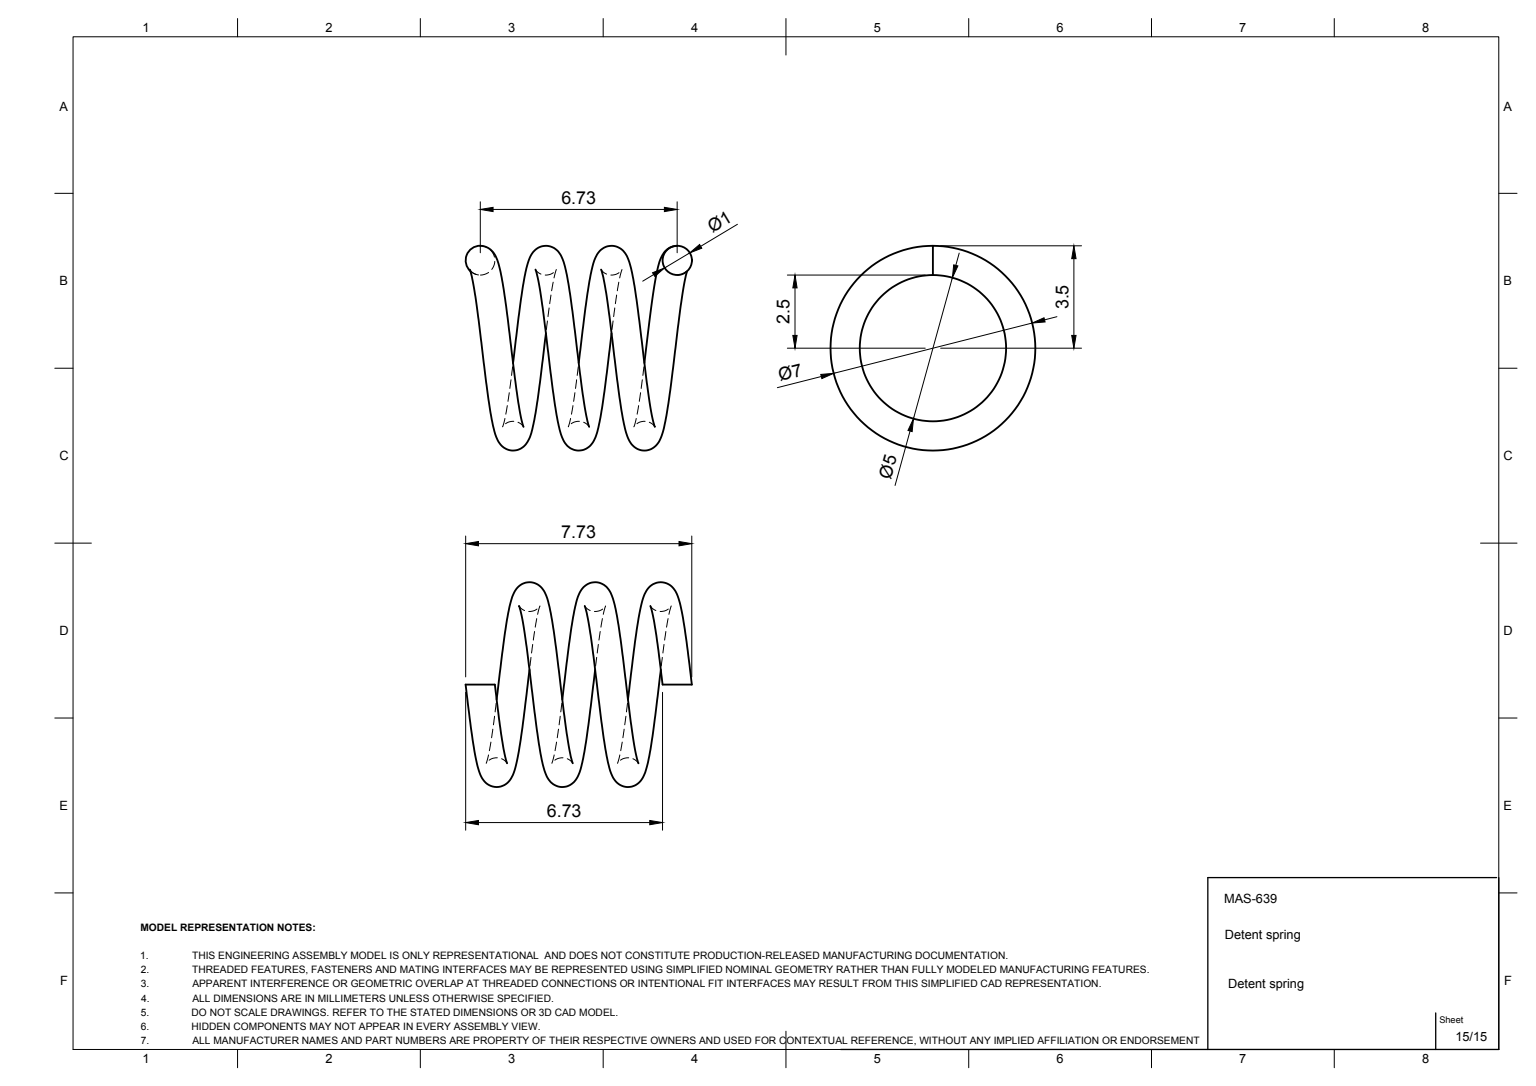
ISO-10303-21;
HEADER;
/* Generated by software containing ST-Developer
 * from STEP Tools, Inc. (www.steptools.com) 
 */

FILE_DESCRIPTION(
/* description */ ('Independent maintained push-to-latch/pull-to-reset mushroom-operator 
CAD. Two opposed spring-loaded ball detents in turned circular seats b
ias both travel stops; direct normally-closed bridge opens6mm when pre
ssed. Rounded palm/pull rim, captured head screw, removable detent clo
sures, native Coil spring families, insulated shared terminals and ord
inary machining features. Manual geometric states and ideal same-mater
ial spring-energy direction only; no electrical/safety certification, 
force/contact dynamics, wear, load or life rating. Requested blue/gray
 visual palette, not safety identification. External wiring/anchors an
d application engineering omitted.'),
/* implementation_level */ '2;1');

FILE_NAME(
/* name */ 'Detent spring.step',
/* time_stamp */ '2026-11-08T17:54:26-08:00',
/* author */ (''),
/* organization */ (''),
/* preprocessor_version */ 'ST-DEVELOPER v20.2',
/* originating_system */ 'Autodesk Translation Framework v15.17.0.0',
/* authorisation */ '');

FILE_SCHEMA (('AUTOMOTIVE_DESIGN { 1 0 10303 214 3 1 1 }'));
ENDSEC;

DATA;
#10=MECHANICAL_DESIGN_GEOMETRIC_PRESENTATION_REPRESENTATION('',(#202),#43980);
#168=SHAPE_REPRESENTATION_RELATIONSHIP('SRR','None',#44068,#185);
#185=ADVANCED_BREP_SHAPE_REPRESENTATION('',(#219),#43975);
#202=STYLED_ITEM('',(#44155),#219);
#219=MANIFOLD_SOLID_BREP('Body1',#11243);
#249=B_SPLINE_SURFACE_WITH_KNOTS('',3,3,((#35913,#35914,#35915,#35916,#35917,
#35918,#35919,#35920,#35921,#35922,#35923,#35924,#35925,#35926,#35927,#35928,
#35929,#35930,#35931,#35932,#35933,#35934,#35935,#35936,#35937,#35938,#35939,
#35940,#35941,#35942,#35943,#35944,#35945,#35946,#35947,#35948,#35949,#35950,
#35951,#35952,#35953),(#35954,#35955,#35956,#35957,#35958,#35959,#35960,
#35961,#35962,#35963,#35964,#35965,#35966,#35967,#35968,#35969,#35970,#35971,
#35972,#35973,#35974,#35975,#35976,#35977,#35978,#35979,#35980,#35981,#35982,
#35983,#35984,#35985,#35986,#35987,#35988,#35989,#35990,#35991,#35992,#35993,
#35994),(#35995,#35996,#35997,#35998,#35999,#36000,#36001,#36002,#36003,
#36004,#36005,#36006,#36007,#36008,#36009,#36010,#36011,#36012,#36013,#36014,
#36015,#36016,#36017,#36018,#36019,#36020,#36021,#36022,#36023,#36024,#36025,
#36026,#36027,#36028,#36029,#36030,#36031,#36032,#36033,#36034,#36035),
(#36036,#36037,#36038,#36039,#36040,#36041,#36042,#36043,#36044,#36045,
#36046,#36047,#36048,#36049,#36050,#36051,#36052,#36053,#36054,#36055,#36056,
#36057,#36058,#36059,#36060,#36061,#36062,#36063,#36064,#36065,#36066,#36067,
#36068,#36069,#36070,#36071,#36072,#36073,#36074,#36075,#36076),(#36077,
#36078,#36079,#36080,#36081,#36082,#36083,#36084,#36085,#36086,#36087,#36088,
#36089,#36090,#36091,#36092,#36093,#36094,#36095,#36096,#36097,#36098,#36099,
#36100,#36101,#36102,#36103,#36104,#36105,#36106,#36107,#36108,#36109,#36110,
#36111,#36112,#36113,#36114,#36115,#36116,#36117),(#36118,#36119,#36120,
#36121,#36122,#36123,#36124,#36125,#36126,#36127,#36128,#36129,#36130,#36131,
#36132,#36133,#36134,#36135,#36136,#36137,#36138,#36139,#36140,#36141,#36142,
#36143,#36144,#36145,#36146,#36147,#36148,#36149,#36150,#36151,#36152,#36153,
#36154,#36155,#36156,#36157,#36158),(#36159,#36160,#36161,#36162,#36163,
#36164,#36165,#36166,#36167,#36168,#36169,#36170,#36171,#36172,#36173,#36174,
#36175,#36176,#36177,#36178,#36179,#36180,#36181,#36182,#36183,#36184,#36185,
#36186,#36187,#36188,#36189,#36190,#36191,#36192,#36193,#36194,#36195,#36196,
#36197,#36198,#36199),(#36200,#36201,#36202,#36203,#36204,#36205,#36206,
#36207,#36208,#36209,#36210,#36211,#36212,#36213,#36214,#36215,#36216,#36217,
#36218,#36219,#36220,#36221,#36222,#36223,#36224,#36225,#36226,#36227,#36228,
#36229,#36230,#36231,#36232,#36233,#36234,#36235,#36236,#36237,#36238,#36239,
#36240),(#36241,#36242,#36243,#36244,#36245,#36246,#36247,#36248,#36249,
#36250,#36251,#36252,#36253,#36254,#36255,#36256,#36257,#36258,#36259,#36260,
#36261,#36262,#36263,#36264,#36265,#36266,#36267,#36268,#36269,#36270,#36271,
#36272,#36273,#36274,#36275,#36276,#36277,#36278,#36279,#36280,#36281),
(#36282,#36283,#36284,#36285,#36286,#36287,#36288,#36289,#36290,#36291,
#36292,#36293,#36294,#36295,#36296,#36297,#36298,#36299,#36300,#36301,#36302,
#36303,#36304,#36305,#36306,#36307,#36308,#36309,#36310,#36311,#36312,#36313,
#36314,#36315,#36316,#36317,#36318,#36319,#36320,#36321,#36322)),
 .UNSPECIFIED.,.T.,.F.,.F.,(4,1,1,1,1,1,1,4),(4,1,1,1,1,1,1,1,1,1,1,1,1,
1,1,1,1,1,1,1,1,1,1,1,1,1,1,1,1,1,1,1,1,1,1,1,1,1,4),(-3.14159265358979,
-2.24399475256414,-1.34639685153848,-0.448798950512828,0.448798950512828,
1.34639685153848,2.24399475256414,3.14159265358979),(0.,0.496040945303652,
0.992081890607303,1.48812283591095,1.98416378121461,2.48020472651826,2.97624567182191,
3.47228661712556,3.96832756242921,4.46436850773286,4.96040945303652,5.45645039834017,
5.95249134364382,6.44853228894747,6.94457323425112,7.44061417955477,7.93665512485842,
8.43269607016208,8.92873701546573,9.42477796076938,9.92081890607303,10.4168598513767,
10.9129007966803,11.408941741984,11.9049826872876,12.4010236325913,12.8970645778949,
13.3931055231986,13.8891464685022,14.3851874138059,14.8812283591095,15.3772693044132,
15.8733102497168,16.3693511950205,16.8653921403242,17.3614330856278,17.8574740309315,
18.3535149762351,18.8495559215388),.UNSPECIFIED.);
#442=PLANE('',#12051);
#443=PLANE('',#12052);
#947=FACE_OUTER_BOUND('',#1634,.T.);
#948=FACE_OUTER_BOUND('',#1635,.T.);
#949=FACE_OUTER_BOUND('',#1636,.T.);
#1634=EDGE_LOOP('',(#9337,#9338,#9339,#9340));
#1635=EDGE_LOOP('',(#9341));
#1636=EDGE_LOOP('',(#9342));
#1962=CIRCLE('',#12049,0.05);
#1963=CIRCLE('',#12050,0.05);
#2609=B_SPLINE_CURVE_WITH_KNOTS('',3,(#36326,#36327,#36328,#36329,#36330,
#36331,#36332,#36333,#36334,#36335,#36336,#36337,#36338,#36339,#36340,#36341,
#36342,#36343,#36344,#36345,#36346,#36347,#36348,#36349,#36350,#36351,#36352,
#36353,#36354,#36355,#36356,#36357,#36358,#36359,#36360,#36361,#36362,#36363,
#36364,#36365,#36366),.UNSPECIFIED.,.F.,.F.,(4,1,1,1,1,1,1,1,1,1,1,1,1,
1,1,1,1,1,1,1,1,1,1,1,1,1,1,1,1,1,1,1,1,1,1,1,1,1,4),(0.,0.496040945303652,
0.992081890607303,1.48812283591095,1.98416378121461,2.48020472651826,2.97624567182191,
3.47228661712556,3.96832756242921,4.46436850773286,4.96040945303652,5.45645039834017,
5.95249134364382,6.44853228894747,6.94457323425112,7.44061417955477,7.93665512485842,
8.43269607016208,8.92873701546573,9.42477796076938,9.92081890607303,10.4168598513767,
10.9129007966803,11.408941741984,11.9049826872876,12.4010236325913,12.8970645778949,
13.3931055231986,13.8891464685022,14.3851874138059,14.8812283591095,15.3772693044132,
15.8733102497168,16.3693511950205,16.8653921403242,17.3614330856278,17.8574740309315,
18.3535149762351,18.8495559215388),.UNSPECIFIED.);
#4918=VERTEX_POINT('',#36323);
#4919=VERTEX_POINT('',#36325);
#6438=EDGE_CURVE('',#4918,#4918,#1962,.T.);
#6439=EDGE_CURVE('',#4918,#4919,#2609,.T.);
#6440=EDGE_CURVE('',#4919,#4919,#1963,.T.);
#9337=ORIENTED_EDGE('',*,*,#6438,.T.);
#9338=ORIENTED_EDGE('',*,*,#6439,.T.);
#9339=ORIENTED_EDGE('',*,*,#6440,.F.);
#9340=ORIENTED_EDGE('',*,*,#6439,.F.);
#9341=ORIENTED_EDGE('',*,*,#6440,.T.);
#9342=ORIENTED_EDGE('',*,*,#6438,.F.);
#11072=ADVANCED_FACE('',(#947),#249,.T.);
#11073=ADVANCED_FACE('',(#948),#442,.F.);
#11074=ADVANCED_FACE('',(#949),#443,.T.);
#11243=CLOSED_SHELL('',(#11072,#11073,#11074));
#12048=AXIS2_PLACEMENT_3D('',#35912,#13951,#13952);
#12049=AXIS2_PLACEMENT_3D('',#36324,#13953,#13954);
#12050=AXIS2_PLACEMENT_3D('',#36367,#13955,#13956);
#12051=AXIS2_PLACEMENT_3D('',#36368,#13957,#13958);
#12052=AXIS2_PLACEMENT_3D('',#36369,#13959,#13960);
#13951=DIRECTION('axis',(0.,0.,1.));
#13952=DIRECTION('refdir',(1.,0.,0.));
#13953=DIRECTION('center_axis',(0.,0.,-1.));
#13954=DIRECTION('ref_axis',(-1.,0.,0.));
#13955=DIRECTION('center_axis',(7.34788079488412E-16,0.,-1.));
#13956=DIRECTION('ref_axis',(-1.,0.,-7.34788079488412E-16));
#13957=DIRECTION('center_axis',(-7.34788079488412E-16,0.,1.));
#13958=DIRECTION('ref_axis',(1.,0.,7.34788079488412E-16));
#13959=DIRECTION('center_axis',(0.,0.,1.));
#13960=DIRECTION('ref_axis',(1.,0.,0.));
#35912=CARTESIAN_POINT('',(0.,0.,0.));
#35913=CARTESIAN_POINT('Ctrl Pts',(0.35,-6.12323399573676E-18,0.));
#35914=CARTESIAN_POINT('Ctrl Pts',(0.35,0.00590530772593761,-0.0578714436187594));
#35915=CARTESIAN_POINT('Ctrl Pts',(0.320737036978914,0.0177159231778128,
-0.173548309605457));
#35916=CARTESIAN_POINT('Ctrl Pts',(0.199460245847326,0.0354318463556257,
-0.305323295892745));
#35917=CARTESIAN_POINT('Ctrl Pts',(0.0301195604177668,0.0531477695334385,
-0.363416175774699));
#35918=CARTESIAN_POINT('Ctrl Pts',(-0.146502340124411,0.0708636927112515,
-0.333985996548453));
#35919=CARTESIAN_POINT('Ctrl Pts',(-0.287770405730312,0.088579615889064,
-0.223981002451209));
#35920=CARTESIAN_POINT('Ctrl Pts',(-0.359728502950795,0.106295539066877,
-0.0600284421673934));
#35921=CARTESIAN_POINT('Ctrl Pts',(-0.344906058802126,0.12401146224469,
0.118406781736645));
#35922=CARTESIAN_POINT('Ctrl Pts',(-0.247005954023888,0.141727385422503,
0.268319590417229));
#35923=CARTESIAN_POINT('Ctrl Pts',(-0.0895198614025972,0.159443308600316,
0.353506441262074));
#35924=CARTESIAN_POINT('Ctrl Pts',(0.0895288995299922,0.177159231778128,
0.353541847300449));
#35925=CARTESIAN_POINT('Ctrl Pts',(0.246980934267327,0.194875154955941,
0.268292799062886));
#35926=CARTESIAN_POINT('Ctrl Pts',(0.344941099461226,0.212591078133754,
0.118418424896554));
#35927=CARTESIAN_POINT('Ctrl Pts',(0.359691482037638,0.230307001311567,
-0.0600218865157286));
#35928=CARTESIAN_POINT('Ctrl Pts',(0.287800848035351,0.248022924489379,
-0.22400439780941));
#35929=CARTESIAN_POINT('Ctrl Pts',(0.146484276133641,0.265738847667193,
-0.33395050615258));
#35930=CARTESIAN_POINT('Ctrl Pts',(-0.0301168255445678,0.283454770845005,
-0.363456018331913));
#35931=CARTESIAN_POINT('Ctrl Pts',(-0.199452865725669,0.301170694022818,
-0.305285338376046));
#35932=CARTESIAN_POINT('Ctrl Pts',(-0.320745536260988,0.318886617200631,
-0.173578803829894));
#35933=CARTESIAN_POINT('Ctrl Pts',(-0.364665029422868,0.336602540378444,
-2.32705416708787E-16));
#35934=CARTESIAN_POINT('Ctrl Pts',(-0.320745536260988,0.354318463556256,
0.173578803829895));
#35935=CARTESIAN_POINT('Ctrl Pts',(-0.199452865725669,0.37203438673407,
0.305285338376046));
#35936=CARTESIAN_POINT('Ctrl Pts',(-0.0301168255445679,0.389750309911882,
0.363456018331913));
#35937=CARTESIAN_POINT('Ctrl Pts',(0.146484276133641,0.407466233089696,
0.33395050615258));
#35938=CARTESIAN_POINT('Ctrl Pts',(0.287800848035351,0.425182156267507,
0.224004397809409));
#35939=CARTESIAN_POINT('Ctrl Pts',(0.359691482037638,0.442898079445321,
0.0600218865157286));
#35940=CARTESIAN_POINT('Ctrl Pts',(0.344941099461226,0.460614002623134,
-0.118418424896554));
#35941=CARTESIAN_POINT('Ctrl Pts',(0.246980934267327,0.478329925800947,
-0.268292799062886));
#35942=CARTESIAN_POINT('Ctrl Pts',(0.0895288995299929,0.49604584897876,
-0.353541847300449));
#35943=CARTESIAN_POINT('Ctrl Pts',(-0.0895198614025975,0.513761772156572,
-0.353506441262075));
#35944=CARTESIAN_POINT('Ctrl Pts',(-0.247005954023888,0.531477695334385,
-0.268319590417228));
#35945=CARTESIAN_POINT('Ctrl Pts',(-0.344906058802126,0.549193618512198,
-0.118406781736645));
#35946=CARTESIAN_POINT('Ctrl Pts',(-0.359728502950795,0.56690954169001,
0.0600284421673935));
#35947=CARTESIAN_POINT('Ctrl Pts',(-0.287770405730312,0.584625464867824,
0.223981002451209));
#35948=CARTESIAN_POINT('Ctrl Pts',(-0.146502340124411,0.602341388045636,
0.333985996548453));
#35949=CARTESIAN_POINT('Ctrl Pts',(0.0301195604177669,0.62005731122345,
0.3634161757747));
#35950=CARTESIAN_POINT('Ctrl Pts',(0.199460245847326,0.637773234401262,
0.305323295892745));
#35951=CARTESIAN_POINT('Ctrl Pts',(0.320737036978914,0.655489157579075,
0.173548309605457));
#35952=CARTESIAN_POINT('Ctrl Pts',(0.35,0.66729977303095,0.0578714436187596));
#35953=CARTESIAN_POINT('Ctrl Pts',(0.35,0.673205080756888,2.57175827820944E-16));
#35954=CARTESIAN_POINT('Ctrl Pts',(0.35,-0.0149599650170943,0.));
#35955=CARTESIAN_POINT('Ctrl Pts',(0.35,-0.00905465729115664,-0.0578939412128541));
#35956=CARTESIAN_POINT('Ctrl Pts',(0.320737127540777,0.00275595816071859,
-0.17353420038403));
#35957=CARTESIAN_POINT('Ctrl Pts',(0.199462254474698,0.0204718813385314,
-0.305334734920036));
#35958=CARTESIAN_POINT('Ctrl Pts',(0.0301198482341514,0.0381878045163443,
-0.363411053172193));
#35959=CARTESIAN_POINT('Ctrl Pts',(-0.146504814797102,0.0559037276941571,
-0.33399283744356));
#35960=CARTESIAN_POINT('Ctrl Pts',(-0.287768683388874,0.0736196508719699,
-0.223978927605389));
#35961=CARTESIAN_POINT('Ctrl Pts',(-0.359733999999531,0.0913355740497829,
-0.060029831390249));
#35962=CARTESIAN_POINT('Ctrl Pts',(-0.344904107829491,0.109051497227595,
0.118406345723654));
#35963=CARTESIAN_POINT('Ctrl Pts',(-0.247009698820708,0.126767420405409,
0.268323507761981));
#35964=CARTESIAN_POINT('Ctrl Pts',(-0.0895193547402367,0.144483343583221,
0.353504534892372));
#35965=CARTESIAN_POINT('Ctrl Pts',(0.0895302448190081,0.162199266761034,
0.353547145096981));
#35966=CARTESIAN_POINT('Ctrl Pts',(0.246979562985841,0.179915189938847,
0.268291322927849));
#35967=CARTESIAN_POINT('Ctrl Pts',(0.344946301010151,0.19763111311666,0.118420201706933));
#35968=CARTESIAN_POINT('Ctrl Pts',(0.35968948216843,0.215347036294473,-0.0600215483887705));
#35969=CARTESIAN_POINT('Ctrl Pts',(0.287805188713831,0.233062959472285,
-0.224007779090794));
#35970=CARTESIAN_POINT('Ctrl Pts',(0.14648346160033,0.250778882650098,-0.333948647665377));
#35971=CARTESIAN_POINT('Ctrl Pts',(-0.0301172799130791,0.268494805827911,
-0.363461501186809));
#35972=CARTESIAN_POINT('Ctrl Pts',(-0.199451756376582,0.286210729005724,
-0.305283640177881));
#35973=CARTESIAN_POINT('Ctrl Pts',(-0.320750374264358,0.303926652183536,
-0.173581422140521));
#35974=CARTESIAN_POINT('Ctrl Pts',(-0.364663001235008,0.32164257536135,
-2.44953070219776E-16));
#35975=CARTESIAN_POINT('Ctrl Pts',(-0.320750374264359,0.339358498539162,
0.173581422140521));
#35976=CARTESIAN_POINT('Ctrl Pts',(-0.199451756376583,0.357074421716976,
0.305283640177881));
#35977=CARTESIAN_POINT('Ctrl Pts',(-0.0301172799130792,0.374790344894787,
0.363461501186809));
#35978=CARTESIAN_POINT('Ctrl Pts',(0.14648346160033,0.392506268072602,0.333948647665377));
#35979=CARTESIAN_POINT('Ctrl Pts',(0.287805188713831,0.410222191250413,
0.224007779090794));
#35980=CARTESIAN_POINT('Ctrl Pts',(0.35968948216843,0.427938114428227,0.0600215483887707));
#35981=CARTESIAN_POINT('Ctrl Pts',(0.344946301010151,0.445654037606039,
-0.118420201706934));
#35982=CARTESIAN_POINT('Ctrl Pts',(0.246979562985841,0.463369960783852,
-0.268291322927849));
#35983=CARTESIAN_POINT('Ctrl Pts',(0.0895302448190086,0.481085883961665,
-0.353547145096981));
#35984=CARTESIAN_POINT('Ctrl Pts',(-0.0895193547402369,0.498801807139478,
-0.353504534892371));
#35985=CARTESIAN_POINT('Ctrl Pts',(-0.247009698820707,0.516517730317291,
-0.268323507761982));
#35986=CARTESIAN_POINT('Ctrl Pts',(-0.344904107829491,0.534233653495103,
-0.118406345723654));
#35987=CARTESIAN_POINT('Ctrl Pts',(-0.359733999999531,0.551949576672917,
0.0600298313902493));
#35988=CARTESIAN_POINT('Ctrl Pts',(-0.287768683388874,0.569665499850729,
0.223978927605389));
#35989=CARTESIAN_POINT('Ctrl Pts',(-0.146504814797102,0.587381423028543,
0.333992837443561));
#35990=CARTESIAN_POINT('Ctrl Pts',(0.0301198482341516,0.605097346206355,
0.363411053172192));
#35991=CARTESIAN_POINT('Ctrl Pts',(0.199462254474698,0.622813269384167,
0.305334734920036));
#35992=CARTESIAN_POINT('Ctrl Pts',(0.320737127540777,0.640529192561981,
0.17353420038403));
#35993=CARTESIAN_POINT('Ctrl Pts',(0.35,0.652339808013856,0.0578939412128544));
#35994=CARTESIAN_POINT('Ctrl Pts',(0.35,0.658245115739793,2.57175827820944E-16));
#35995=CARTESIAN_POINT('Ctrl Pts',(0.335708111401436,-0.0447458605757917,
0.));
#35996=CARTESIAN_POINT('Ctrl Pts',(0.335708111401436,-0.0388405528498541,
-0.0554977928230549));
#35997=CARTESIAN_POINT('Ctrl Pts',(0.307640028870999,-0.0270299373979789,
-0.166468247501657));
#35998=CARTESIAN_POINT('Ctrl Pts',(0.191314552514196,-0.00931401422016608,
-0.292850380259684));
#35999=CARTESIAN_POINT('Ctrl Pts',(0.0288895245544089,0.00840190895764677,
-0.348578849160588));
#36000=CARTESIAN_POINT('Ctrl Pts',(-0.140518910052752,0.0261178321354596,
-0.32034482131761));
#36001=CARTESIAN_POINT('Ctrl Pts',(-0.276020404510637,0.0438337553132723,
-0.214835940639136));
#36002=CARTESIAN_POINT('Ctrl Pts',(-0.345036788048542,0.0615496784910853,
-0.0575765924801678));
#36003=CARTESIAN_POINT('Ctrl Pts',(-0.330823089198529,0.0792656016688981,
0.113571967147225));
#36004=CARTESIAN_POINT('Ctrl Pts',(-0.236917968165966,0.0969815248467109,
0.257361203462888));
#36005=CARTESIAN_POINT('Ctrl Pts',(-0.0858646474450097,0.114697448024524,
0.339072263044565));
#36006=CARTESIAN_POINT('Ctrl Pts',(0.0858724496913478,0.132413371202337,
0.33910285135484));
#36007=CARTESIAN_POINT('Ctrl Pts',(0.236896364680631,0.150129294380149,
0.257338030560792));
#36008=CARTESIAN_POINT('Ctrl Pts',(0.330853351222059,0.167845217557962,
0.113582099143669));
#36009=CARTESIAN_POINT('Ctrl Pts',(0.34500478782966,0.185561140735775,-0.0575711130196162));
#36010=CARTESIAN_POINT('Ctrl Pts',(0.276046765897809,0.203277063913588,
-0.214855826894537));
#36011=CARTESIAN_POINT('Ctrl Pts',(0.140503123221668,0.220992987091401,
-0.320314851940556));
#36012=CARTESIAN_POINT('Ctrl Pts',(-0.0288868234010755,0.238708910269214,
-0.348612100831537));
#36013=CARTESIAN_POINT('Ctrl Pts',(-0.191308933142308,0.256424833447026,
-0.292820121666851));
#36014=CARTESIAN_POINT('Ctrl Pts',(-0.307645959021329,0.274140756624839,
-0.166489667090601));
#36015=CARTESIAN_POINT('Ctrl Pts',(-0.349775258797716,0.291856679802652,
-1.83714802664832E-16));
#36016=CARTESIAN_POINT('Ctrl Pts',(-0.307645959021329,0.309572602980465,
0.166489667090601));
#36017=CARTESIAN_POINT('Ctrl Pts',(-0.191308933142307,0.327288526158277,
0.292820121666851));
#36018=CARTESIAN_POINT('Ctrl Pts',(-0.0288868234010758,0.345004449336091,
0.348612100831537));
#36019=CARTESIAN_POINT('Ctrl Pts',(0.140503123221668,0.362720372513903,
0.320314851940556));
#36020=CARTESIAN_POINT('Ctrl Pts',(0.27604676589781,0.380436295691716,0.214855826894537));
#36021=CARTESIAN_POINT('Ctrl Pts',(0.34500478782966,0.398152218869529,0.0575711130196162));
#36022=CARTESIAN_POINT('Ctrl Pts',(0.330853351222058,0.415868142047341,
-0.113582099143669));
#36023=CARTESIAN_POINT('Ctrl Pts',(0.236896364680631,0.433584065225155,
-0.257338030560792));
#36024=CARTESIAN_POINT('Ctrl Pts',(0.0858724496913482,0.451299988402968,
-0.33910285135484));
#36025=CARTESIAN_POINT('Ctrl Pts',(-0.0858646474450095,0.46901591158078,
-0.339072263044565));
#36026=CARTESIAN_POINT('Ctrl Pts',(-0.236917968165967,0.486731834758593,
-0.257361203462888));
#36027=CARTESIAN_POINT('Ctrl Pts',(-0.330823089198529,0.504447757936406,
-0.113571967147225));
#36028=CARTESIAN_POINT('Ctrl Pts',(-0.345036788048542,0.522163681114218,
0.0575765924801677));
#36029=CARTESIAN_POINT('Ctrl Pts',(-0.276020404510636,0.539879604292032,
0.214835940639137));
#36030=CARTESIAN_POINT('Ctrl Pts',(-0.140518910052752,0.557595527469844,
0.320344821317609));
#36031=CARTESIAN_POINT('Ctrl Pts',(0.0288895245544092,0.575311450647657,
0.348578849160589));
#36032=CARTESIAN_POINT('Ctrl Pts',(0.191314552514196,0.59302737382547,0.292850380259683));
#36033=CARTESIAN_POINT('Ctrl Pts',(0.307640028870999,0.610743297003283,
0.166468247501657));
#36034=CARTESIAN_POINT('Ctrl Pts',(0.335708111401436,0.622553912455158,
0.0554977928230551));
#36035=CARTESIAN_POINT('Ctrl Pts',(0.335708111401436,0.628459220181096,
2.46674318445343E-16));
#36036=CARTESIAN_POINT('Ctrl Pts',(0.287271575555009,-0.0557889266101467,
0.));
#36037=CARTESIAN_POINT('Ctrl Pts',(0.287271575555009,-0.0498836188842091,
-0.0475015952121335));
#36038=CARTESIAN_POINT('Ctrl Pts',(0.263253248344736,-0.0380730034323339,
-0.142442953697593));
#36039=CARTESIAN_POINT('Ctrl Pts',(0.163712356953626,-0.020357080254521,
-0.250603083626219));
#36040=CARTESIAN_POINT('Ctrl Pts',(0.0247214371762577,-0.00264115707670821,
-0.298282769894969));
#36041=CARTESIAN_POINT('Ctrl Pts',(-0.120245826277052,0.0150747661011046,
-0.27412830773178));
#36042=CARTESIAN_POINT('Ctrl Pts',(-0.236194861111183,0.0327906892789176,
-0.183838021283139));
#36043=CARTESIAN_POINT('Ctrl Pts',(-0.295257011496817,0.0505066124567302,
-0.0492700305779588));
#36044=CARTESIAN_POINT('Ctrl Pts',(-0.283090408491503,0.0682225356345432,
0.0971853955774754));
#36045=CARTESIAN_POINT('Ctrl Pts',(-0.202736892426251,0.0859384588123559,
0.220230628323799));
#36046=CARTESIAN_POINT('Ctrl Pts',(-0.0734757000535192,0.103654381990169,
0.290149399582528));
#36047=CARTESIAN_POINT('Ctrl Pts',(0.0734832917947263,0.121370305167982,
0.290179134787802));
#36048=CARTESIAN_POINT('Ctrl Pts',(0.202715877612707,0.139086228345794,
0.220208133442515));
#36049=CARTESIAN_POINT('Ctrl Pts',(0.283119838964945,0.156802151523607,
0.0971951592678911));
#36050=CARTESIAN_POINT('Ctrl Pts',(0.295225923420481,0.17451807470142,-0.0492644880639345));
#36051=CARTESIAN_POINT('Ctrl Pts',(0.236220415317673,0.192233997879233,
-0.183857734680427));
#36052=CARTESIAN_POINT('Ctrl Pts',(0.120230691703391,0.209949921057046,
-0.274098363237872));
#36053=CARTESIAN_POINT('Ctrl Pts',(-0.0247192080583375,0.227665844234859,
-0.298316465071458));
#36054=CARTESIAN_POINT('Ctrl Pts',(-0.16370600748086,0.245381767412672,
-0.250570698506515));
#36055=CARTESIAN_POINT('Ctrl Pts',(-0.263260669021949,0.263097690590484,
-0.142469549414193));
#36056=CARTESIAN_POINT('Ctrl Pts',(-0.299308088749296,0.280813613768297,
4.89906140439551E-17));
#36057=CARTESIAN_POINT('Ctrl Pts',(-0.263260669021949,0.29852953694611,
0.142469549414192));
#36058=CARTESIAN_POINT('Ctrl Pts',(-0.163706007480861,0.316245460123924,
0.250570698506515));
#36059=CARTESIAN_POINT('Ctrl Pts',(-0.0247192080583377,0.333961383301735,
0.298316465071458));
#36060=CARTESIAN_POINT('Ctrl Pts',(0.120230691703391,0.351677306479549,
0.274098363237873));
#36061=CARTESIAN_POINT('Ctrl Pts',(0.236220415317673,0.369393229657361,
0.183857734680427));
#36062=CARTESIAN_POINT('Ctrl Pts',(0.295225923420481,0.387109152835174,
0.0492644880639345));
#36063=CARTESIAN_POINT('Ctrl Pts',(0.283119838964945,0.404825076012987,
-0.0971951592678911));
#36064=CARTESIAN_POINT('Ctrl Pts',(0.202715877612707,0.4225409991908,-0.220208133442515));
#36065=CARTESIAN_POINT('Ctrl Pts',(0.0734832917947267,0.440256922368613,
-0.290179134787802));
#36066=CARTESIAN_POINT('Ctrl Pts',(-0.0734757000535193,0.457972845546425,
-0.290149399582527));
#36067=CARTESIAN_POINT('Ctrl Pts',(-0.202736892426251,0.47568876872424,
-0.220230628323799));
#36068=CARTESIAN_POINT('Ctrl Pts',(-0.283090408491504,0.493404691902051,
-0.0971853955774754));
#36069=CARTESIAN_POINT('Ctrl Pts',(-0.295257011496816,0.511120615079865,
0.0492700305779587));
#36070=CARTESIAN_POINT('Ctrl Pts',(-0.236194861111183,0.528836538257677,
0.183838021283139));
#36071=CARTESIAN_POINT('Ctrl Pts',(-0.120245826277051,0.54655246143549,
0.27412830773178));
#36072=CARTESIAN_POINT('Ctrl Pts',(0.0247214371762577,0.564268384613303,
0.298282769894969));
#36073=CARTESIAN_POINT('Ctrl Pts',(0.163712356953627,0.581984307791115,
0.250603083626218));
#36074=CARTESIAN_POINT('Ctrl Pts',(0.263253248344736,0.599700230968929,
0.142442953697593));
#36075=CARTESIAN_POINT('Ctrl Pts',(0.287271575555009,0.611510846420803,
0.0475015952121336));
#36076=CARTESIAN_POINT('Ctrl Pts',(0.287271575555009,0.617416154146741,
2.11083729293675E-16));
#36077=CARTESIAN_POINT('Ctrl Pts',(0.2483964525207,-0.0248377821418625,
0.));
#36078=CARTESIAN_POINT('Ctrl Pts',(0.2483964525207,-0.0189324744159249,
-0.0410748300994032));
#36079=CARTESIAN_POINT('Ctrl Pts',(0.227628419209138,-0.00712185896404963,
-0.123165932150964));
#36080=CARTESIAN_POINT('Ctrl Pts',(0.141558052308102,0.0105940642137631,
-0.216690850682477));
#36081=CARTESIAN_POINT('Ctrl Pts',(0.0213760183023638,0.0283099873915761,
-0.257917233510476));
#36082=CARTESIAN_POINT('Ctrl Pts',(-0.103973673673943,0.0460259105693889,
-0.237032228868884));
#36083=CARTESIAN_POINT('Ctrl Pts',(-0.204231604209003,0.0637418337472016,
-0.158959949419166));
#36084=CARTESIAN_POINT('Ctrl Pts',(-0.255301599773748,0.0814577569250147,
-0.0426026337570547));
#36085=CARTESIAN_POINT('Ctrl Pts',(-0.244780981522273,0.0991736801028273,
0.0840337218647635));
#36086=CARTESIAN_POINT('Ctrl Pts',(-0.175301687703595,0.11688960328064,
0.190428088650001));
#36087=CARTESIAN_POINT('Ctrl Pts',(-0.063532544489394,0.134605526458453,
0.250884715042728));
#36088=CARTESIAN_POINT('Ctrl Pts',(0.0635392244753556,0.152321449636266,
0.250910876008833));
#36089=CARTESIAN_POINT('Ctrl Pts',(0.175283197378719,0.170037372814079,
0.190408301232517));
#36090=CARTESIAN_POINT('Ctrl Pts',(0.244806875770799,0.187753295991892,
0.0840423024059766));
#36091=CARTESIAN_POINT('Ctrl Pts',(0.255274250740611,0.205469219169704,
-0.0425977334636045));
#36092=CARTESIAN_POINT('Ctrl Pts',(0.204254078740494,0.223185142347517,
-0.158977335668398));
#36093=CARTESIAN_POINT('Ctrl Pts',(0.103960381877751,0.24090106552533,-0.23700579360409));
#36094=CARTESIAN_POINT('Ctrl Pts',(-0.0213741012368434,0.258616988703143,
-0.25794703087359));
#36095=CARTESIAN_POINT('Ctrl Pts',(-0.141552367454289,0.276332911880956,
-0.216662028058088));
#36096=CARTESIAN_POINT('Ctrl Pts',(-0.227635132018289,0.294048835058769,
-0.123189972933852));
#36097=CARTESIAN_POINT('Ctrl Pts',(-0.25880399389923,0.311764758236581,
-1.22476535109888E-17));
#36098=CARTESIAN_POINT('Ctrl Pts',(-0.227635132018289,0.329480681414395,
0.123189972933851));
#36099=CARTESIAN_POINT('Ctrl Pts',(-0.141552367454289,0.347196604592207,
0.216662028058088));
#36100=CARTESIAN_POINT('Ctrl Pts',(-0.0213741012368437,0.364912527770019,
0.257947030873589));
#36101=CARTESIAN_POINT('Ctrl Pts',(0.103960381877751,0.382628450947834,
0.23700579360409));
#36102=CARTESIAN_POINT('Ctrl Pts',(0.204254078740494,0.400344374125644,
0.158977335668397));
#36103=CARTESIAN_POINT('Ctrl Pts',(0.255274250740611,0.418060297303459,
0.0425977334636048));
#36104=CARTESIAN_POINT('Ctrl Pts',(0.244806875770799,0.435776220481271,
-0.0840423024059769));
#36105=CARTESIAN_POINT('Ctrl Pts',(0.175283197378719,0.453492143659084,
-0.190408301232516));
#36106=CARTESIAN_POINT('Ctrl Pts',(0.0635392244753558,0.471208066836898,
-0.250910876008834));
#36107=CARTESIAN_POINT('Ctrl Pts',(-0.063532544489394,0.488923990014709,
-0.250884715042728));
#36108=CARTESIAN_POINT('Ctrl Pts',(-0.175301687703595,0.506639913192522,
-0.190428088650001));
#36109=CARTESIAN_POINT('Ctrl Pts',(-0.244780981522273,0.524355836370335,
-0.0840337218647634));
#36110=CARTESIAN_POINT('Ctrl Pts',(-0.255301599773748,0.542071759548147,
0.0426026337570547));
#36111=CARTESIAN_POINT('Ctrl Pts',(-0.204231604209003,0.559787682725961,
0.158959949419166));
#36112=CARTESIAN_POINT('Ctrl Pts',(-0.103973673673943,0.577503605903774,
0.237032228868883));
#36113=CARTESIAN_POINT('Ctrl Pts',(0.0213760183023641,0.595219529081586,
0.257917233510476));
#36114=CARTESIAN_POINT('Ctrl Pts',(0.141558052308102,0.6129354522594,0.216690850682477));
#36115=CARTESIAN_POINT('Ctrl Pts',(0.227628419209138,0.630651375437212,
0.123165932150964));
#36116=CARTESIAN_POINT('Ctrl Pts',(0.2483964525207,0.642461990889088,0.0410748300994034));
#36117=CARTESIAN_POINT('Ctrl Pts',(0.2483964525207,0.648367298615025,1.8251875229942E-16));
#36118=CARTESIAN_POINT('Ctrl Pts',(0.248462856117505,0.024811377463635,
0.));
#36119=CARTESIAN_POINT('Ctrl Pts',(0.248462856117505,0.0307166851895726,
-0.0410773426135567));
#36120=CARTESIAN_POINT('Ctrl Pts',(0.227689236819528,0.0425273006414479,
-0.123204168627986));
#36121=CARTESIAN_POINT('Ctrl Pts',(0.141595138855583,0.0602432238192606,
-0.216744472856645));
#36122=CARTESIAN_POINT('Ctrl Pts',(0.0213816244011575,0.0779591469970735,
-0.257988110411106));
#36123=CARTESIAN_POINT('Ctrl Pts',(-0.104000537406664,0.0956750701748862,
-0.237093019599219));
#36124=CARTESIAN_POINT('Ctrl Pts',(-0.204286849538004,0.113390993352699,
-0.159003224998934));
#36125=CARTESIAN_POINT('Ctrl Pts',(-0.255367780255422,0.131106916530512,
-0.042613499783648));
#36126=CARTESIAN_POINT('Ctrl Pts',(-0.244847152934927,0.148822839708325,
0.08405635063601));
#36127=CARTESIAN_POINT('Ctrl Pts',(-0.175347141420753,0.166538762886138,
0.190477521147925));
#36128=CARTESIAN_POINT('Ctrl Pts',(-0.0635497192916874,0.184254686063951,
0.250952501372567));
#36129=CARTESIAN_POINT('Ctrl Pts',(0.0635557039981047,0.201970609241763,
0.250975957719874));
#36130=CARTESIAN_POINT('Ctrl Pts',(0.175330571819336,0.219686532419577,
0.19045975851969));
#36131=CARTESIAN_POINT('Ctrl Pts',(0.244870361932152,0.237402455597388,
0.0840641005753268));
#36132=CARTESIAN_POINT('Ctrl Pts',(0.255343245713768,0.255118378775203,
-0.0426092483460967));
#36133=CARTESIAN_POINT('Ctrl Pts',(0.20430704798701,0.272834301953014,-0.159018562236839));
#36134=CARTESIAN_POINT('Ctrl Pts',(0.103988480097989,0.290550225130828,
-0.2370698516718));
#36135=CARTESIAN_POINT('Ctrl Pts',(-0.0213796441337567,0.30826614830864,
-0.258013923898435));
#36136=CARTESIAN_POINT('Ctrl Pts',(-0.141590626072894,0.325982071486454,
-0.216720587313536));
#36137=CARTESIAN_POINT('Ctrl Pts',(-0.227694164509807,0.343697994664265,
-0.123221919677699));
#36138=CARTESIAN_POINT('Ctrl Pts',(-0.258873943134403,0.361413917842079,
-7.34859210659327E-17));
#36139=CARTESIAN_POINT('Ctrl Pts',(-0.227694164509807,0.379129841019892,
0.123221919677698));
#36140=CARTESIAN_POINT('Ctrl Pts',(-0.141590626072894,0.396845764197705,
0.216720587313536));
#36141=CARTESIAN_POINT('Ctrl Pts',(-0.0213796441337568,0.414561687375517,
0.258013923898435));
#36142=CARTESIAN_POINT('Ctrl Pts',(0.103988480097989,0.432277610553331,
0.2370698516718));
#36143=CARTESIAN_POINT('Ctrl Pts',(0.20430704798701,0.449993533731143,0.159018562236839));
#36144=CARTESIAN_POINT('Ctrl Pts',(0.255343245713769,0.467709456908956,
0.0426092483460965));
#36145=CARTESIAN_POINT('Ctrl Pts',(0.244870361932151,0.485425380086769,
-0.0840641005753267));
#36146=CARTESIAN_POINT('Ctrl Pts',(0.175330571819337,0.503141303264581,
-0.19045975851969));
#36147=CARTESIAN_POINT('Ctrl Pts',(0.063555703998105,0.520857226442395,
-0.250975957719874));
#36148=CARTESIAN_POINT('Ctrl Pts',(-0.0635497192916875,0.538573149620206,
-0.250952501372567));
#36149=CARTESIAN_POINT('Ctrl Pts',(-0.175347141420753,0.556289072798021,
-0.190477521147925));
#36150=CARTESIAN_POINT('Ctrl Pts',(-0.244847152934927,0.574004995975833,
-0.0840563506360099));
#36151=CARTESIAN_POINT('Ctrl Pts',(-0.255367780255422,0.591720919153647,
0.0426134997836479));
#36152=CARTESIAN_POINT('Ctrl Pts',(-0.204286849538004,0.609436842331458,
0.159003224998935));
#36153=CARTESIAN_POINT('Ctrl Pts',(-0.104000537406664,0.627152765509273,
0.23709301959922));
#36154=CARTESIAN_POINT('Ctrl Pts',(0.0213816244011575,0.644868688687084,
0.257988110411106));
#36155=CARTESIAN_POINT('Ctrl Pts',(0.141595138855583,0.662584611864898,
0.216744472856645));
#36156=CARTESIAN_POINT('Ctrl Pts',(0.227689236819528,0.680300535042709,
0.123204168627986));
#36157=CARTESIAN_POINT('Ctrl Pts',(0.248462856117505,0.692111150494585,
0.0410773426135568));
#36158=CARTESIAN_POINT('Ctrl Pts',(0.248462856117505,0.698016458220523,
1.82567544870787E-16));
#36159=CARTESIAN_POINT('Ctrl Pts',(0.28724245097485,0.055853598532737,0.));
#36160=CARTESIAN_POINT('Ctrl Pts',(0.28724245097485,0.0617589062586746,
-0.0475027005302338));
#36161=CARTESIAN_POINT('Ctrl Pts',(0.263226582660364,0.0735695217105498,
-0.142424798902927));
#36162=CARTESIAN_POINT('Ctrl Pts',(0.163696287887152,0.0912854448883627,
-0.250580687287576));
#36163=CARTESIAN_POINT('Ctrl Pts',(0.0247190065829995,0.109001368066176,
-0.298251180732612));
#36164=CARTESIAN_POINT('Ctrl Pts',(-0.120234286656455,0.126717291243988,
-0.274102316132114));
#36165=CARTESIAN_POINT('Ctrl Pts',(-0.236170461556994,0.144433214421801,
-0.183818837068975));
#36166=CARTESIAN_POINT('Ctrl Pts',(-0.295228524106512,0.162149137599614,
-0.0492654010455716));
#36167=CARTESIAN_POINT('Ctrl Pts',(-0.283061194331496,0.179865060777427,
0.0971754278326294));
#36168=CARTESIAN_POINT('Ctrl Pts',(-0.20271732386458,0.197580983955239,
0.220209331600313));
#36169=CARTESIAN_POINT('Ctrl Pts',(-0.0734681174847661,0.215296907133053,
0.290119481496877));
#36170=CARTESIAN_POINT('Ctrl Pts',(0.0734761958756083,0.233012830310865,
0.290151109768457));
#36171=CARTESIAN_POINT('Ctrl Pts',(0.202694964669258,0.250728753488678,
0.220185419477375));
#36172=CARTESIAN_POINT('Ctrl Pts',(0.283092504309657,0.268444676666491,
0.0971857729312045));
#36173=CARTESIAN_POINT('Ctrl Pts',(0.295195466051039,0.286160599844304,
-0.0492594044683245));
#36174=CARTESIAN_POINT('Ctrl Pts',(0.236197608912768,0.303876523022116,
-0.18383998447823));
#36175=CARTESIAN_POINT('Ctrl Pts',(0.120218287923552,0.32159244619993,-0.274070085063785));
#36176=CARTESIAN_POINT('Ctrl Pts',(-0.0247168215263096,0.339308369377742,
-0.298287663767521));
#36177=CARTESIAN_POINT('Ctrl Pts',(-0.163689118430773,0.357024292555555,
-0.25054484783482));
#36178=CARTESIAN_POINT('Ctrl Pts',(-0.263235252075215,0.374740215733368,
-0.142455794480522));
#36179=CARTESIAN_POINT('Ctrl Pts',(-0.299277210062645,0.392456138911181,
-1.22476535109888E-17));
#36180=CARTESIAN_POINT('Ctrl Pts',(-0.263235252075215,0.410172062088994,
0.142455794480522));
#36181=CARTESIAN_POINT('Ctrl Pts',(-0.163689118430773,0.427887985266806,
0.250544847834821));
#36182=CARTESIAN_POINT('Ctrl Pts',(-0.0247168215263098,0.445603908444619,
0.29828766376752));
#36183=CARTESIAN_POINT('Ctrl Pts',(0.120218287923551,0.463319831622433,
0.274070085063786));
#36184=CARTESIAN_POINT('Ctrl Pts',(0.236197608912768,0.481035754800244,
0.18383998447823));
#36185=CARTESIAN_POINT('Ctrl Pts',(0.29519546605104,0.498751677978058,0.0492594044683247));
#36186=CARTESIAN_POINT('Ctrl Pts',(0.283092504309657,0.51646760115587,-0.0971857729312049));
#36187=CARTESIAN_POINT('Ctrl Pts',(0.202694964669258,0.534183524333684,
-0.220185419477374));
#36188=CARTESIAN_POINT('Ctrl Pts',(0.0734761958756085,0.551899447511496,
-0.290151109768457));
#36189=CARTESIAN_POINT('Ctrl Pts',(-0.073468117484766,0.569615370689309,
-0.290119481496877));
#36190=CARTESIAN_POINT('Ctrl Pts',(-0.20271732386458,0.587331293867122,
-0.220209331600313));
#36191=CARTESIAN_POINT('Ctrl Pts',(-0.283061194331496,0.605047217044934,
-0.0971754278326294));
#36192=CARTESIAN_POINT('Ctrl Pts',(-0.295228524106513,0.622763140222748,
0.0492654010455718));
#36193=CARTESIAN_POINT('Ctrl Pts',(-0.236170461556994,0.64047906340056,
0.183818837068975));
#36194=CARTESIAN_POINT('Ctrl Pts',(-0.120234286656455,0.658194986578373,
0.274102316132114));
#36195=CARTESIAN_POINT('Ctrl Pts',(0.0247190065829998,0.675910909756186,
0.298251180732612));
#36196=CARTESIAN_POINT('Ctrl Pts',(0.163696287887152,0.693626832933998,
0.250580687287576));
#36197=CARTESIAN_POINT('Ctrl Pts',(0.263226582660364,0.711342756111813,
0.142424798902927));
#36198=CARTESIAN_POINT('Ctrl Pts',(0.28724245097485,0.723153371563687,0.047502700530234));
#36199=CARTESIAN_POINT('Ctrl Pts',(0.28724245097485,0.729058679289624,2.11062328899355E-16));
#36200=CARTESIAN_POINT('Ctrl Pts',(0.335700057265398,0.0447030440973884,
0.));
#36201=CARTESIAN_POINT('Ctrl Pts',(0.335700057265398,0.050608351823326,
-0.0554935013777734));
#36202=CARTESIAN_POINT('Ctrl Pts',(0.307632636214863,0.0624189672752012,
-0.166466110007902));
#36203=CARTESIAN_POINT('Ctrl Pts',(0.191309698322281,0.0801348904530141,
-0.292841849330558));
#36204=CARTESIAN_POINT('Ctrl Pts',(0.0288887935843006,0.0978508136308268,
-0.348571160208687));
#36205=CARTESIAN_POINT('Ctrl Pts',(-0.140515213206916,0.11556673680864,
-0.320336235724583));
#36206=CARTESIAN_POINT('Ctrl Pts',(-0.276014008976892,0.133282659986453,
-0.214831059389936));
#36207=CARTESIAN_POINT('Ctrl Pts',(-0.345027786866192,0.150998583164266,
-0.0575750283544988));
#36208=CARTESIAN_POINT('Ctrl Pts',(-0.330815408947634,0.168714506342078,
0.113569299752606));
#36209=CARTESIAN_POINT('Ctrl Pts',(-0.236911791455489,0.186430429519891,
0.257354513587));
#36210=CARTESIAN_POINT('Ctrl Pts',(-0.0858626540853489,0.204146352697704,
0.339064379015408));
#36211=CARTESIAN_POINT('Ctrl Pts',(0.0858702124863541,0.221862275875517,
0.33909401875172));
#36212=CARTESIAN_POINT('Ctrl Pts',(0.23689086160232,0.23957819905333,0.257332050851972));
#36213=CARTESIAN_POINT('Ctrl Pts',(0.330844729199832,0.257294122231142,
0.113579140368498));
#36214=CARTESIAN_POINT('Ctrl Pts',(0.344996773771998,0.275010045408956,
-0.0575697762899338));
#36215=CARTESIAN_POINT('Ctrl Pts',(0.276039572030225,0.292725968586768,
-0.214850227314705));
#36216=CARTESIAN_POINT('Ctrl Pts',(0.140499859509914,0.310441891764581,
-0.32030741162972));
#36217=CARTESIAN_POINT('Ctrl Pts',(-0.0288860705827872,0.328157814942394,
-0.348603015739585));
#36218=CARTESIAN_POINT('Ctrl Pts',(-0.191304489312158,0.345873738120207,
-0.292813319906457));
#36219=CARTESIAN_POINT('Ctrl Pts',(-0.30763794160998,0.363589661298019,
-0.166485328269541));
#36220=CARTESIAN_POINT('Ctrl Pts',(-0.349767134015211,0.381305584475832,
-1.22476535109888E-16));
#36221=CARTESIAN_POINT('Ctrl Pts',(-0.30763794160998,0.399021507653645,
0.166485328269541));
#36222=CARTESIAN_POINT('Ctrl Pts',(-0.191304489312158,0.416737430831458,
0.292813319906457));
#36223=CARTESIAN_POINT('Ctrl Pts',(-0.0288860705827875,0.43445335400927,
0.348603015739585));
#36224=CARTESIAN_POINT('Ctrl Pts',(0.140499859509914,0.452169277187084,
0.320307411629721));
#36225=CARTESIAN_POINT('Ctrl Pts',(0.276039572030225,0.469885200364896,
0.214850227314704));
#36226=CARTESIAN_POINT('Ctrl Pts',(0.344996773771998,0.487601123542709,
0.0575697762899342));
#36227=CARTESIAN_POINT('Ctrl Pts',(0.330844729199832,0.505317046720522,
-0.113579140368499));
#36228=CARTESIAN_POINT('Ctrl Pts',(0.23689086160232,0.523032969898335,-0.257332050851972));
#36229=CARTESIAN_POINT('Ctrl Pts',(0.0858702124863545,0.540748893076148,
-0.339094018751721));
#36230=CARTESIAN_POINT('Ctrl Pts',(-0.0858626540853487,0.55846481625396,
-0.339064379015408));
#36231=CARTESIAN_POINT('Ctrl Pts',(-0.23691179145549,0.576180739431775,
-0.257354513587));
#36232=CARTESIAN_POINT('Ctrl Pts',(-0.330815408947634,0.593896662609586,
-0.113569299752606));
#36233=CARTESIAN_POINT('Ctrl Pts',(-0.345027786866192,0.611612585787399,
0.0575750283544989));
#36234=CARTESIAN_POINT('Ctrl Pts',(-0.276014008976891,0.629328508965212,
0.214831059389936));
#36235=CARTESIAN_POINT('Ctrl Pts',(-0.140515213206917,0.647044432143026,
0.320336235724583));
#36236=CARTESIAN_POINT('Ctrl Pts',(0.028888793584301,0.664760355320838,
0.348571160208686));
#36237=CARTESIAN_POINT('Ctrl Pts',(0.191309698322281,0.682476278498651,
0.292841849330559));
#36238=CARTESIAN_POINT('Ctrl Pts',(0.307632636214863,0.700192201676463,
0.166466110007902));
#36239=CARTESIAN_POINT('Ctrl Pts',(0.335700057265398,0.712002817128339,
0.0554935013777736));
#36240=CARTESIAN_POINT('Ctrl Pts',(0.335700057265398,0.717908124854276,
2.46668400362192E-16));
#36241=CARTESIAN_POINT('Ctrl Pts',(0.35,0.0149599650170943,0.));
#36242=CARTESIAN_POINT('Ctrl Pts',(0.35,0.0208652727430319,-0.0578968747192045));
#36243=CARTESIAN_POINT('Ctrl Pts',(0.32073713934932,0.0326758881949071,
-0.173532360654391));
#36244=CARTESIAN_POINT('Ctrl Pts',(0.199462516383644,0.0503918113727199,
-0.305336226477714));
#36245=CARTESIAN_POINT('Ctrl Pts',(0.0301198857631062,0.0681077345505328,
-0.363410385225793));
#36246=CARTESIAN_POINT('Ctrl Pts',(-0.14650513747463,0.0858236577283456,
-0.333993729441574));
#36247=CARTESIAN_POINT('Ctrl Pts',(-0.287768458809325,0.103539580906158,
-0.223978657062087));
#36248=CARTESIAN_POINT('Ctrl Pts',(-0.359734716770725,0.121255504083971,
-0.0600300125337997));
#36249=CARTESIAN_POINT('Ctrl Pts',(-0.344903853438262,0.138971427261784,
0.118406288871047));
#36250=CARTESIAN_POINT('Ctrl Pts',(-0.247010187112264,0.156687350439597,
0.268324018552409));
#36251=CARTESIAN_POINT('Ctrl Pts',(-0.089519288675517,0.174403273617409,
0.353504286317008));
#36252=CARTESIAN_POINT('Ctrl Pts',(0.0895304202339372,0.192119196795223,
0.353547835887281));
#36253=CARTESIAN_POINT('Ctrl Pts',(0.246979384181701,0.209835119973035,
0.268291130451645));
#36254=CARTESIAN_POINT('Ctrl Pts',(0.344946979250533,0.227551043150848,
0.118420433388797));
#36255=CARTESIAN_POINT('Ctrl Pts',(0.359689221401479,0.245266966328661,
-0.0600215042997194));
#36256=CARTESIAN_POINT('Ctrl Pts',(0.287805754703591,0.262982889506474,
-0.224008219982846));
#36257=CARTESIAN_POINT('Ctrl Pts',(0.1464833553917,0.280698812684287,-0.333948405333508));
#36258=CARTESIAN_POINT('Ctrl Pts',(-0.0301173391590991,0.298414735862099,
-0.36346221610724));
#36259=CARTESIAN_POINT('Ctrl Pts',(-0.199451611726333,0.316130659039913,
-0.305283418746421));
#36260=CARTESIAN_POINT('Ctrl Pts',(-0.320751005101307,0.333846582217725,
-0.173581763547288));
#36261=CARTESIAN_POINT('Ctrl Pts',(-0.36466273677553,0.351562505395538,
-1.59219495642854E-16));
#36262=CARTESIAN_POINT('Ctrl Pts',(-0.320751005101307,0.369278428573351,
0.173581763547288));
#36263=CARTESIAN_POINT('Ctrl Pts',(-0.199451611726333,0.386994351751164,
0.305283418746421));
#36264=CARTESIAN_POINT('Ctrl Pts',(-0.0301173391590995,0.404710274928977,
0.36346221610724));
#36265=CARTESIAN_POINT('Ctrl Pts',(0.1464833553917,0.422426198106789,0.333948405333509));
#36266=CARTESIAN_POINT('Ctrl Pts',(0.28780575470359,0.440142121284602,0.224008219982845));
#36267=CARTESIAN_POINT('Ctrl Pts',(0.359689221401479,0.457858044462415,
0.0600215042997194));
#36268=CARTESIAN_POINT('Ctrl Pts',(0.344946979250532,0.475573967640229,
-0.118420433388797));
#36269=CARTESIAN_POINT('Ctrl Pts',(0.246979384181702,0.49328989081804,-0.268291130451645));
#36270=CARTESIAN_POINT('Ctrl Pts',(0.0895304202339372,0.511005813995854,
-0.353547835887281));
#36271=CARTESIAN_POINT('Ctrl Pts',(-0.0895192886755167,0.528721737173666,
-0.353504286317008));
#36272=CARTESIAN_POINT('Ctrl Pts',(-0.247010187112265,0.54643766035148,
-0.268324018552409));
#36273=CARTESIAN_POINT('Ctrl Pts',(-0.344903853438262,0.564153583529292,
-0.118406288871046));
#36274=CARTESIAN_POINT('Ctrl Pts',(-0.359734716770725,0.581869506707105,
0.0600300125337994));
#36275=CARTESIAN_POINT('Ctrl Pts',(-0.287768458809324,0.599585429884918,
0.223978657062087));
#36276=CARTESIAN_POINT('Ctrl Pts',(-0.14650513747463,0.617301353062731,
0.333993729441574));
#36277=CARTESIAN_POINT('Ctrl Pts',(0.0301198857631064,0.635017276240543,
0.363410385225793));
#36278=CARTESIAN_POINT('Ctrl Pts',(0.199462516383644,0.652733199418356,
0.305336226477713));
#36279=CARTESIAN_POINT('Ctrl Pts',(0.320737139349319,0.670449122596169,
0.173532360654391));
#36280=CARTESIAN_POINT('Ctrl Pts',(0.35,0.682259738048044,0.0578968747192047));
#36281=CARTESIAN_POINT('Ctrl Pts',(0.35,0.688165045773982,2.57175827820944E-16));
#36282=CARTESIAN_POINT('Ctrl Pts',(0.35,6.12323399573676E-18,0.));
#36283=CARTESIAN_POINT('Ctrl Pts',(0.35,0.00590530772593762,-0.0578714436187594));
#36284=CARTESIAN_POINT('Ctrl Pts',(0.320737036978914,0.0177159231778128,
-0.173548309605457));
#36285=CARTESIAN_POINT('Ctrl Pts',(0.199460245847326,0.0354318463556257,
-0.305323295892745));
#36286=CARTESIAN_POINT('Ctrl Pts',(0.0301195604177668,0.0531477695334385,
-0.363416175774699));
#36287=CARTESIAN_POINT('Ctrl Pts',(-0.146502340124411,0.0708636927112515,
-0.333985996548453));
#36288=CARTESIAN_POINT('Ctrl Pts',(-0.287770405730312,0.088579615889064,
-0.223981002451209));
#36289=CARTESIAN_POINT('Ctrl Pts',(-0.359728502950795,0.106295539066877,
-0.0600284421673934));
#36290=CARTESIAN_POINT('Ctrl Pts',(-0.344906058802126,0.12401146224469,
0.118406781736645));
#36291=CARTESIAN_POINT('Ctrl Pts',(-0.247005954023888,0.141727385422503,
0.268319590417229));
#36292=CARTESIAN_POINT('Ctrl Pts',(-0.0895198614025972,0.159443308600316,
0.353506441262074));
#36293=CARTESIAN_POINT('Ctrl Pts',(0.0895288995299922,0.177159231778128,
0.353541847300449));
#36294=CARTESIAN_POINT('Ctrl Pts',(0.246980934267327,0.194875154955941,
0.268292799062886));
#36295=CARTESIAN_POINT('Ctrl Pts',(0.344941099461226,0.212591078133754,
0.118418424896554));
#36296=CARTESIAN_POINT('Ctrl Pts',(0.359691482037638,0.230307001311567,
-0.0600218865157286));
#36297=CARTESIAN_POINT('Ctrl Pts',(0.287800848035351,0.248022924489379,
-0.22400439780941));
#36298=CARTESIAN_POINT('Ctrl Pts',(0.146484276133641,0.265738847667193,
-0.33395050615258));
#36299=CARTESIAN_POINT('Ctrl Pts',(-0.0301168255445678,0.283454770845005,
-0.363456018331913));
#36300=CARTESIAN_POINT('Ctrl Pts',(-0.199452865725669,0.301170694022818,
-0.305285338376046));
#36301=CARTESIAN_POINT('Ctrl Pts',(-0.320745536260988,0.318886617200631,
-0.173578803829894));
#36302=CARTESIAN_POINT('Ctrl Pts',(-0.364665029422868,0.336602540378444,
-2.32705416708787E-16));
#36303=CARTESIAN_POINT('Ctrl Pts',(-0.320745536260988,0.354318463556256,
0.173578803829895));
#36304=CARTESIAN_POINT('Ctrl Pts',(-0.199452865725669,0.37203438673407,
0.305285338376046));
#36305=CARTESIAN_POINT('Ctrl Pts',(-0.0301168255445679,0.389750309911882,
0.363456018331913));
#36306=CARTESIAN_POINT('Ctrl Pts',(0.146484276133641,0.407466233089696,
0.33395050615258));
#36307=CARTESIAN_POINT('Ctrl Pts',(0.287800848035351,0.425182156267507,
0.224004397809409));
#36308=CARTESIAN_POINT('Ctrl Pts',(0.359691482037638,0.442898079445321,
0.0600218865157286));
#36309=CARTESIAN_POINT('Ctrl Pts',(0.344941099461226,0.460614002623134,
-0.118418424896554));
#36310=CARTESIAN_POINT('Ctrl Pts',(0.246980934267327,0.478329925800947,
-0.268292799062886));
#36311=CARTESIAN_POINT('Ctrl Pts',(0.0895288995299929,0.49604584897876,
-0.353541847300449));
#36312=CARTESIAN_POINT('Ctrl Pts',(-0.0895198614025975,0.513761772156572,
-0.353506441262075));
#36313=CARTESIAN_POINT('Ctrl Pts',(-0.247005954023888,0.531477695334385,
-0.268319590417228));
#36314=CARTESIAN_POINT('Ctrl Pts',(-0.344906058802126,0.549193618512198,
-0.118406781736645));
#36315=CARTESIAN_POINT('Ctrl Pts',(-0.359728502950795,0.56690954169001,
0.0600284421673935));
#36316=CARTESIAN_POINT('Ctrl Pts',(-0.287770405730312,0.584625464867824,
0.223981002451209));
#36317=CARTESIAN_POINT('Ctrl Pts',(-0.146502340124411,0.602341388045636,
0.333985996548453));
#36318=CARTESIAN_POINT('Ctrl Pts',(0.0301195604177669,0.62005731122345,
0.3634161757747));
#36319=CARTESIAN_POINT('Ctrl Pts',(0.199460245847326,0.637773234401262,
0.305323295892745));
#36320=CARTESIAN_POINT('Ctrl Pts',(0.320737036978914,0.655489157579075,
0.173548309605457));
#36321=CARTESIAN_POINT('Ctrl Pts',(0.35,0.66729977303095,0.0578714436187596));
#36322=CARTESIAN_POINT('Ctrl Pts',(0.35,0.673205080756888,2.57175827820944E-16));
#36323=CARTESIAN_POINT('',(0.35,-6.12323399573676E-18,0.));
#36324=CARTESIAN_POINT('Origin',(0.3,0.,0.));
#36325=CARTESIAN_POINT('',(0.35,0.673205080756888,2.57175827820944E-16));
#36326=CARTESIAN_POINT('Ctrl Pts',(0.35,6.12323399573676E-18,0.));
#36327=CARTESIAN_POINT('Ctrl Pts',(0.35,0.00590530772593762,-0.0578714436187594));
#36328=CARTESIAN_POINT('Ctrl Pts',(0.320737036978914,0.0177159231778128,
-0.173548309605457));
#36329=CARTESIAN_POINT('Ctrl Pts',(0.199460245847326,0.0354318463556257,
-0.305323295892745));
#36330=CARTESIAN_POINT('Ctrl Pts',(0.0301195604177668,0.0531477695334385,
-0.363416175774699));
#36331=CARTESIAN_POINT('Ctrl Pts',(-0.146502340124411,0.0708636927112515,
-0.333985996548453));
#36332=CARTESIAN_POINT('Ctrl Pts',(-0.287770405730312,0.088579615889064,
-0.223981002451209));
#36333=CARTESIAN_POINT('Ctrl Pts',(-0.359728502950795,0.106295539066877,
-0.0600284421673934));
#36334=CARTESIAN_POINT('Ctrl Pts',(-0.344906058802126,0.12401146224469,
0.118406781736645));
#36335=CARTESIAN_POINT('Ctrl Pts',(-0.247005954023888,0.141727385422503,
0.268319590417229));
#36336=CARTESIAN_POINT('Ctrl Pts',(-0.0895198614025972,0.159443308600316,
0.353506441262074));
#36337=CARTESIAN_POINT('Ctrl Pts',(0.0895288995299922,0.177159231778128,
0.353541847300449));
#36338=CARTESIAN_POINT('Ctrl Pts',(0.246980934267327,0.194875154955941,
0.268292799062886));
#36339=CARTESIAN_POINT('Ctrl Pts',(0.344941099461226,0.212591078133754,
0.118418424896554));
#36340=CARTESIAN_POINT('Ctrl Pts',(0.359691482037638,0.230307001311567,
-0.0600218865157286));
#36341=CARTESIAN_POINT('Ctrl Pts',(0.287800848035351,0.248022924489379,
-0.22400439780941));
#36342=CARTESIAN_POINT('Ctrl Pts',(0.146484276133641,0.265738847667193,
-0.33395050615258));
#36343=CARTESIAN_POINT('Ctrl Pts',(-0.0301168255445678,0.283454770845005,
-0.363456018331913));
#36344=CARTESIAN_POINT('Ctrl Pts',(-0.199452865725669,0.301170694022818,
-0.305285338376046));
#36345=CARTESIAN_POINT('Ctrl Pts',(-0.320745536260988,0.318886617200631,
-0.173578803829894));
#36346=CARTESIAN_POINT('Ctrl Pts',(-0.364665029422868,0.336602540378444,
-2.32705416708787E-16));
#36347=CARTESIAN_POINT('Ctrl Pts',(-0.320745536260988,0.354318463556256,
0.173578803829895));
#36348=CARTESIAN_POINT('Ctrl Pts',(-0.199452865725669,0.37203438673407,
0.305285338376046));
#36349=CARTESIAN_POINT('Ctrl Pts',(-0.0301168255445679,0.389750309911882,
0.363456018331913));
#36350=CARTESIAN_POINT('Ctrl Pts',(0.146484276133641,0.407466233089696,
0.33395050615258));
#36351=CARTESIAN_POINT('Ctrl Pts',(0.287800848035351,0.425182156267507,
0.224004397809409));
#36352=CARTESIAN_POINT('Ctrl Pts',(0.359691482037638,0.442898079445321,
0.0600218865157286));
#36353=CARTESIAN_POINT('Ctrl Pts',(0.344941099461226,0.460614002623134,
-0.118418424896554));
#36354=CARTESIAN_POINT('Ctrl Pts',(0.246980934267327,0.478329925800947,
-0.268292799062886));
#36355=CARTESIAN_POINT('Ctrl Pts',(0.0895288995299929,0.49604584897876,
-0.353541847300449));
#36356=CARTESIAN_POINT('Ctrl Pts',(-0.0895198614025975,0.513761772156572,
-0.353506441262075));
#36357=CARTESIAN_POINT('Ctrl Pts',(-0.247005954023888,0.531477695334385,
-0.268319590417228));
#36358=CARTESIAN_POINT('Ctrl Pts',(-0.344906058802126,0.549193618512198,
-0.118406781736645));
#36359=CARTESIAN_POINT('Ctrl Pts',(-0.359728502950795,0.56690954169001,
0.0600284421673935));
#36360=CARTESIAN_POINT('Ctrl Pts',(-0.287770405730312,0.584625464867824,
0.223981002451209));
#36361=CARTESIAN_POINT('Ctrl Pts',(-0.146502340124411,0.602341388045636,
0.333985996548453));
#36362=CARTESIAN_POINT('Ctrl Pts',(0.0301195604177669,0.62005731122345,
0.3634161757747));
#36363=CARTESIAN_POINT('Ctrl Pts',(0.199460245847326,0.637773234401262,
0.305323295892745));
#36364=CARTESIAN_POINT('Ctrl Pts',(0.320737036978914,0.655489157579075,
0.173548309605457));
#36365=CARTESIAN_POINT('Ctrl Pts',(0.35,0.66729977303095,0.0578714436187596));
#36366=CARTESIAN_POINT('Ctrl Pts',(0.35,0.673205080756888,2.57175827820944E-16));
#36367=CARTESIAN_POINT('Origin',(0.3,0.673205080756888,2.20436423846524E-16));
#36368=CARTESIAN_POINT('Origin',(0.3,0.673205080756888,2.20436423846524E-16));
#36369=CARTESIAN_POINT('Origin',(0.3,7.2280144832367E-19,0.));
#43956=UNCERTAINTY_MEASURE_WITH_UNIT(LENGTH_MEASURE(0.001),#43981,
'DISTANCE_ACCURACY_VALUE',
'Maximum model space distance between geometric entities at asserted c
onnectivities');
#43961=UNCERTAINTY_MEASURE_WITH_UNIT(LENGTH_MEASURE(0.001),#43981,
'DISTANCE_ACCURACY_VALUE',
'Maximum model space distance between geometric entities at asserted c
onnectivities');
#43975=(
GEOMETRIC_REPRESENTATION_CONTEXT(3)
GLOBAL_UNCERTAINTY_ASSIGNED_CONTEXT((#43956))
GLOBAL_UNIT_ASSIGNED_CONTEXT((#43981,#43983,#43984))
REPRESENTATION_CONTEXT('','3D')
);
#43980=(
GEOMETRIC_REPRESENTATION_CONTEXT(3)
GLOBAL_UNCERTAINTY_ASSIGNED_CONTEXT((#43961))
GLOBAL_UNIT_ASSIGNED_CONTEXT((#43981,#43983,#43984))
REPRESENTATION_CONTEXT('','3D')
);
#43981=(
LENGTH_UNIT()
NAMED_UNIT(*)
SI_UNIT(.CENTI.,.METRE.)
);
#43983=(
NAMED_UNIT(*)
PLANE_ANGLE_UNIT()
SI_UNIT($,.RADIAN.)
);
#43984=(
NAMED_UNIT(*)
SI_UNIT($,.STERADIAN.)
SOLID_ANGLE_UNIT()
);
#43998=SHAPE_DEFINITION_REPRESENTATION(#44016,#44068);
#44016=PRODUCT_DEFINITION_SHAPE('',$,#44087);
#44068=SHAPE_REPRESENTATION('',(#12048),#43975);
#44073=PRODUCT_DEFINITION_CONTEXT('part definition',#44129,'design');
#44087=PRODUCT_DEFINITION('Detent spring','Detent spring',#44105,#44073);
#44105=PRODUCT_DEFINITION_FORMATION('',$,#44144);
#44129=APPLICATION_CONTEXT(
'Core Data for Automotive Mechanical Design Process');
#44130=PRODUCT_CONTEXT('part definition',#44129,'mechanical');
#44144=PRODUCT('Detent spring','Detent spring','Detent spring',(#44130));
#44155=PRESENTATION_STYLE_ASSIGNMENT((#44167));
#44167=SURFACE_STYLE_USAGE(.BOTH.,#44179);
#44179=SURFACE_SIDE_STYLE('',(#44191));
#44191=SURFACE_STYLE_FILL_AREA(#44203);
#44203=FILL_AREA_STYLE('Spring gray',(#44215));
#44215=FILL_AREA_STYLE_COLOUR('Spring gray',#44227);
#44227=COLOUR_RGB('Spring gray',0.407843137254902,0.447058823529412,0.498039215686275);
ENDSEC;
END-ISO-10303-21;
